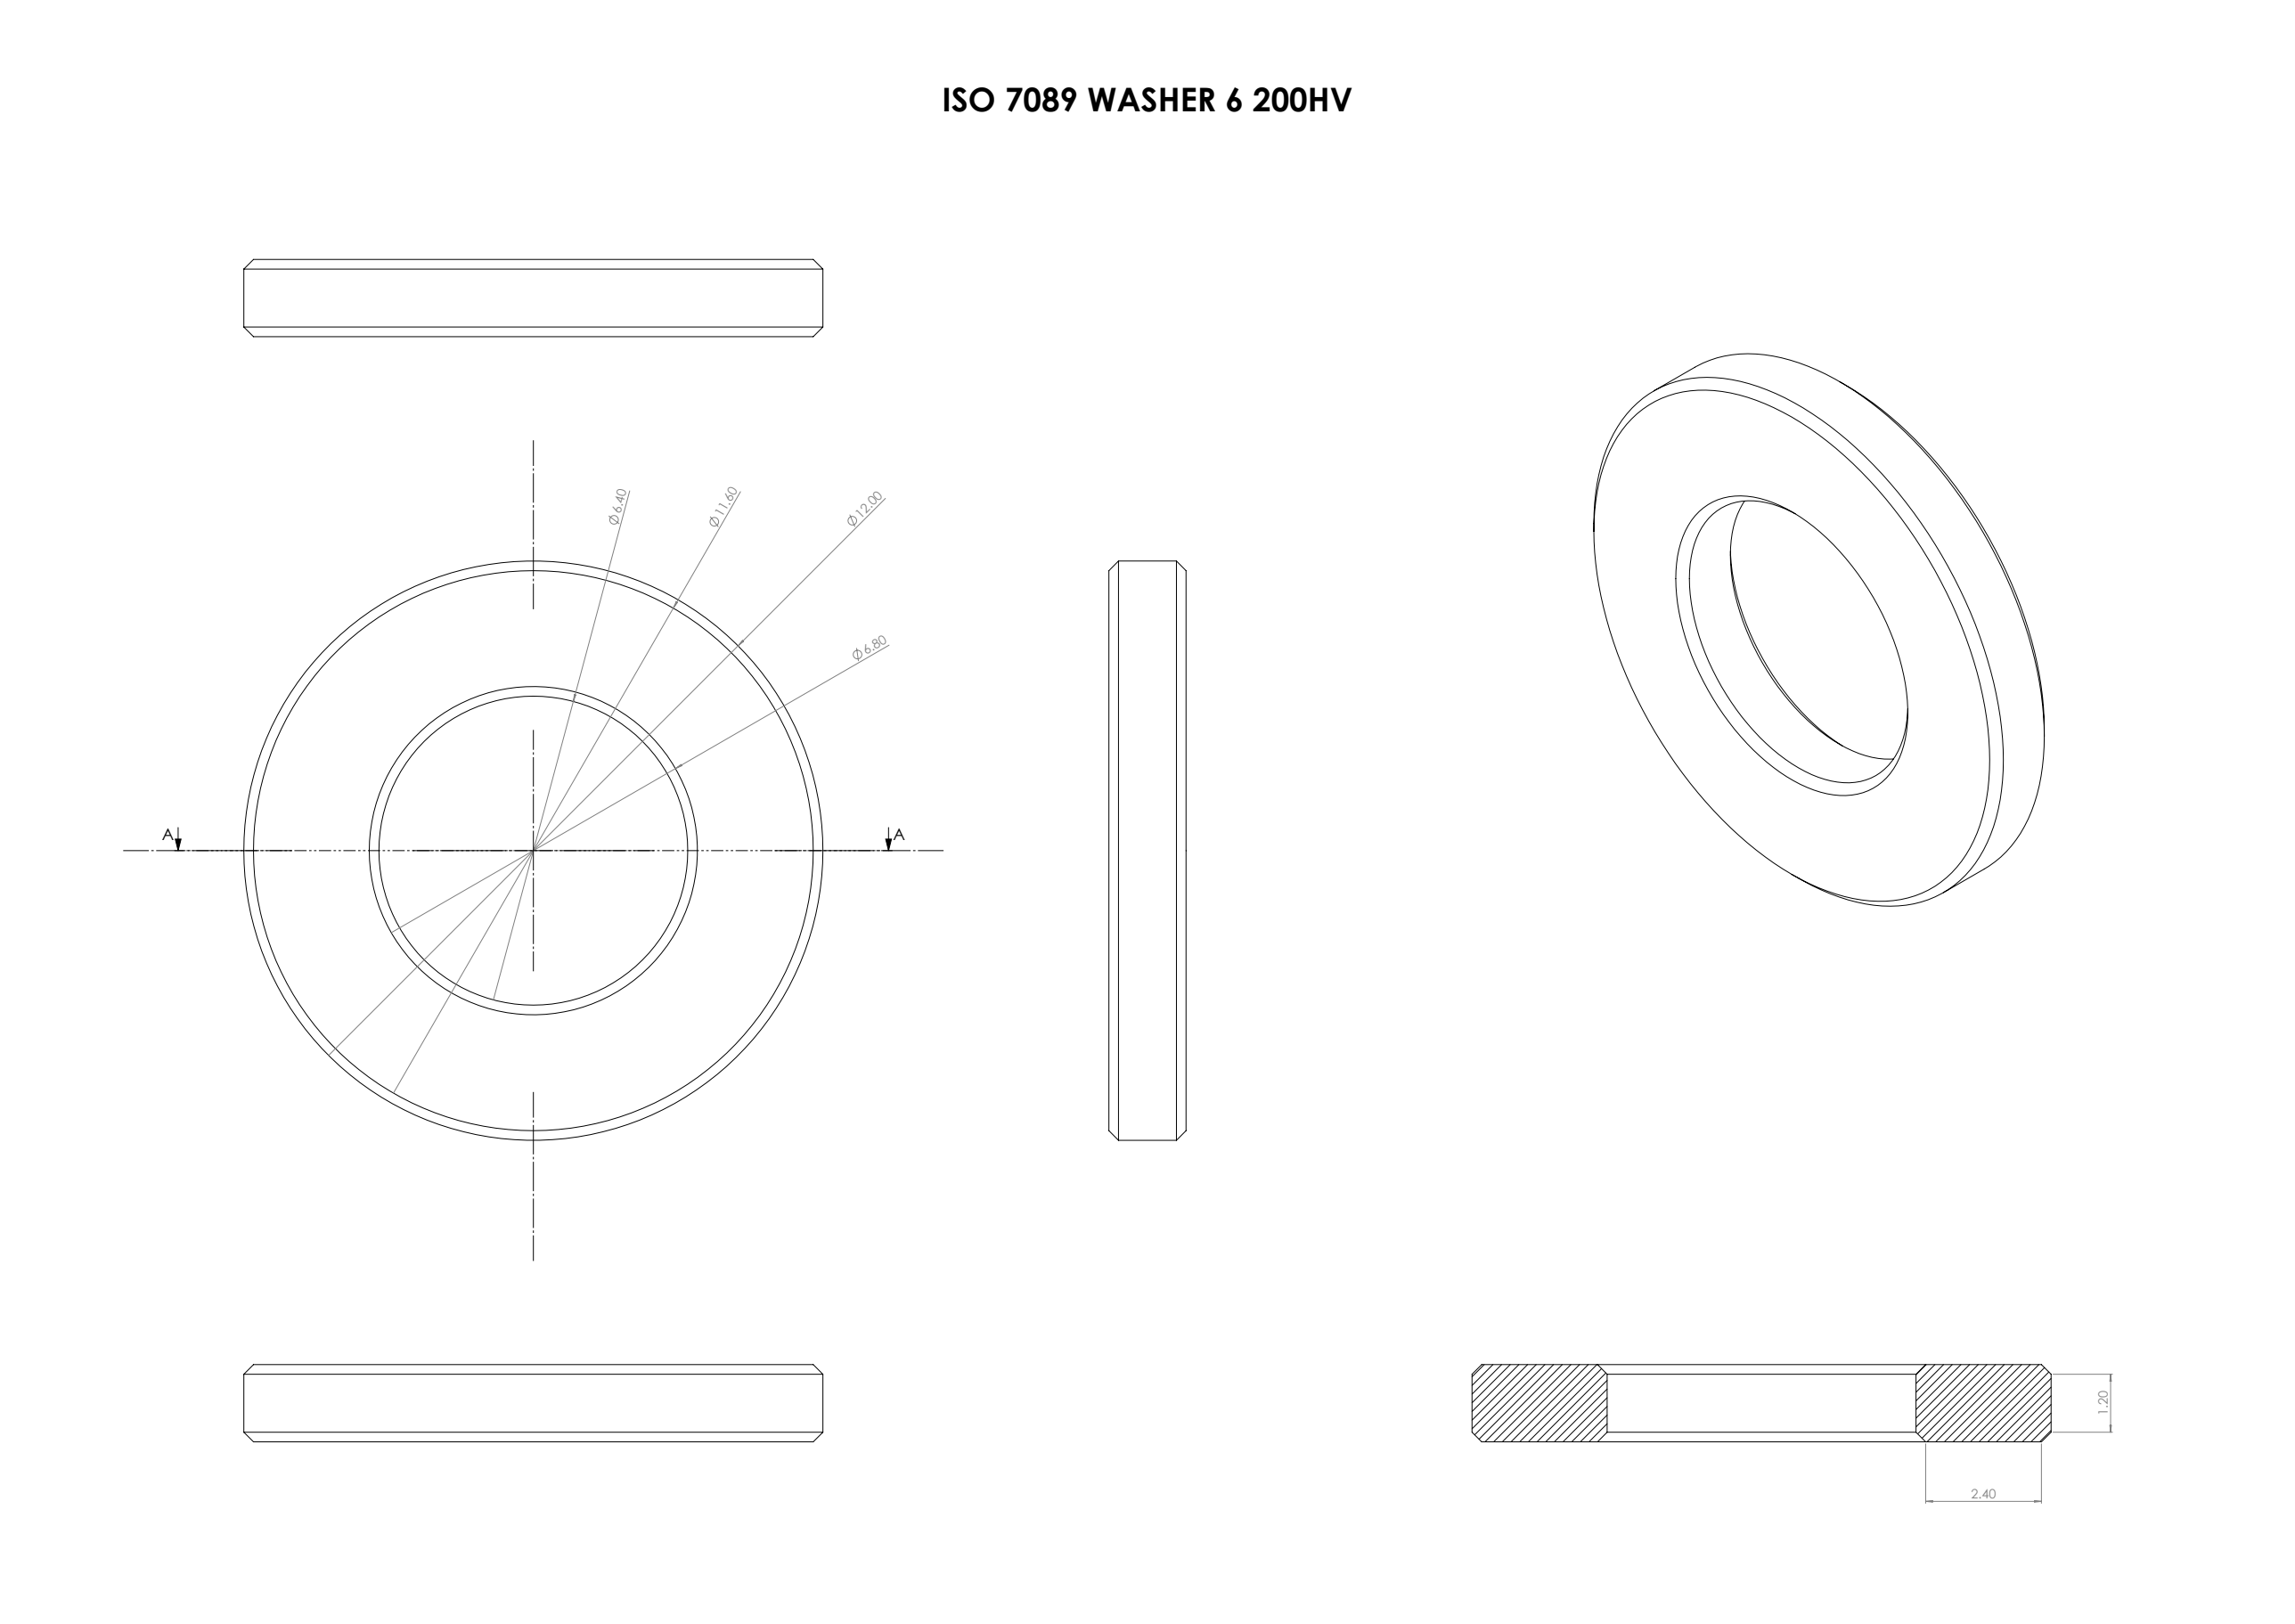
ISO-10303-21;
HEADER;
/* Generated by software containing ST-Developer
 * from STEP Tools, Inc. (www.steptools.com) 
 */

FILE_DESCRIPTION(
/* description */ (''),
/* implementation_level */ '2;1');

FILE_NAME(
/* name */ 
'10_ISO_7089_Washer_6_200HV.step',
/* time_stamp */ '2026-10-22T00:21:42-07:00',
/* author */ (''),
/* organization */ (''),
/* preprocessor_version */ 'ST-DEVELOPER v20.2',
/* originating_system */ 'Autodesk Translation Framework v15.15.0.0',
/* authorisation */ '');

FILE_SCHEMA (('AUTOMOTIVE_DESIGN { 1 0 10303 214 3 1 1 }'));
ENDSEC;

DATA;
#10=MECHANICAL_DESIGN_GEOMETRIC_PRESENTATION_REPRESENTATION('',(#214),#31638);
#192=SHAPE_REPRESENTATION_RELATIONSHIP('SRR','None',#31714,#203);
#203=ADVANCED_BREP_SHAPE_REPRESENTATION('',(#225),#31636);
#214=STYLED_ITEM('',(#31837),#225);
#225=MANIFOLD_SOLID_BREP('Washer',#12489);
#359=CYLINDRICAL_SURFACE('',#13522,0.6);
#360=CYLINDRICAL_SURFACE('',#13528,0.32);
#441=CONICAL_SURFACE('',#13516,0.59,0.785398163397449);
#442=CONICAL_SURFACE('',#13524,0.33,0.785398163397449);
#443=CONICAL_SURFACE('',#13533,0.33,0.785398163397449);
#444=CONICAL_SURFACE('',#13534,0.59,0.785398163397449);
#1401=FACE_BOUND('',#3223,.T.);
#1402=FACE_BOUND('',#3228,.T.);
#1794=CIRCLE('',#13517,0.58);
#1795=CIRCLE('',#13518,0.6);
#1796=CIRCLE('',#13519,0.6);
#1797=CIRCLE('',#13521,0.34);
#1798=CIRCLE('',#13523,0.6);
#1799=CIRCLE('',#13525,0.34);
#1800=CIRCLE('',#13526,0.32);
#1801=CIRCLE('',#13527,0.32);
#1802=CIRCLE('',#13529,0.32);
#1803=CIRCLE('',#13530,0.32);
#1804=CIRCLE('',#13532,0.58);
#2466=FACE_OUTER_BOUND('',#3221,.T.);
#2467=FACE_OUTER_BOUND('',#3222,.T.);
#2468=FACE_OUTER_BOUND('',#3224,.T.);
#2469=FACE_OUTER_BOUND('',#3225,.T.);
#2470=FACE_OUTER_BOUND('',#3226,.T.);
#2471=FACE_OUTER_BOUND('',#3227,.T.);
#2472=FACE_OUTER_BOUND('',#3229,.T.);
#2473=FACE_OUTER_BOUND('',#3230,.T.);
#3221=EDGE_LOOP('',(#11271,#11272,#11273,#11274,#11275));
#3222=EDGE_LOOP('',(#11276));
#3223=EDGE_LOOP('',(#11277));
#3224=EDGE_LOOP('',(#11278,#11279,#11280,#11281,#11282));
#3225=EDGE_LOOP('',(#11283,#11284,#11285,#11286,#11287));
#3226=EDGE_LOOP('',(#11288,#11289,#11290,#11291,#11292,#11293));
#3227=EDGE_LOOP('',(#11294));
#3228=EDGE_LOOP('',(#11295));
#3229=EDGE_LOOP('',(#11296,#11297,#11298,#11299,#11300));
#3230=EDGE_LOOP('',(#11301,#11302,#11303,#11304));
#3946=LINE('',#30956,#4651);
#3947=LINE('',#30965,#4652);
#3948=LINE('',#30971,#4653);
#3949=LINE('',#30980,#4654);
#3950=LINE('',#30985,#4655);
#3951=LINE('',#30987,#4656);
#4651=VECTOR('',#16104,0.59);
#4652=VECTOR('',#16115,0.6);
#4653=VECTOR('',#16122,0.33);
#4654=VECTOR('',#16133,0.32);
#4655=VECTOR('',#16140,0.33);
#4656=VECTOR('',#16143,0.59);
#5825=VERTEX_POINT('',#30953);
#5826=VERTEX_POINT('',#30955);
#5827=VERTEX_POINT('',#30957);
#5828=VERTEX_POINT('',#30961);
#5829=VERTEX_POINT('',#30964);
#5830=VERTEX_POINT('',#30968);
#5831=VERTEX_POINT('',#30970);
#5832=VERTEX_POINT('',#30972);
#5833=VERTEX_POINT('',#30976);
#5834=VERTEX_POINT('',#30977);
#5835=VERTEX_POINT('',#30982);
#7647=EDGE_CURVE('',#5825,#5825,#1794,.T.);
#7648=EDGE_CURVE('',#5825,#5826,#3946,.T.);
#7649=EDGE_CURVE('',#5826,#5827,#1795,.T.);
#7650=EDGE_CURVE('',#5827,#5826,#1796,.T.);
#7651=EDGE_CURVE('',#5828,#5828,#1797,.T.);
#7652=EDGE_CURVE('',#5827,#5829,#3947,.T.);
#7653=EDGE_CURVE('',#5829,#5829,#1798,.T.);
#7654=EDGE_CURVE('',#5830,#5830,#1799,.T.);
#7655=EDGE_CURVE('',#5830,#5831,#3948,.T.);
#7656=EDGE_CURVE('',#5831,#5832,#1800,.T.);
#7657=EDGE_CURVE('',#5832,#5831,#1801,.T.);
#7658=EDGE_CURVE('',#5833,#5834,#1802,.T.);
#7659=EDGE_CURVE('',#5834,#5833,#1803,.T.);
#7660=EDGE_CURVE('',#5834,#5832,#3949,.T.);
#7661=EDGE_CURVE('',#5835,#5835,#1804,.T.);
#7662=EDGE_CURVE('',#5833,#5828,#3950,.T.);
#7663=EDGE_CURVE('',#5829,#5835,#3951,.T.);
#11271=ORIENTED_EDGE('',*,*,#7647,.T.);
#11272=ORIENTED_EDGE('',*,*,#7648,.T.);
#11273=ORIENTED_EDGE('',*,*,#7649,.T.);
#11274=ORIENTED_EDGE('',*,*,#7650,.T.);
#11275=ORIENTED_EDGE('',*,*,#7648,.F.);
#11276=ORIENTED_EDGE('',*,*,#7647,.F.);
#11277=ORIENTED_EDGE('',*,*,#7651,.F.);
#11278=ORIENTED_EDGE('',*,*,#7649,.F.);
#11279=ORIENTED_EDGE('',*,*,#7650,.F.);
#11280=ORIENTED_EDGE('',*,*,#7652,.T.);
#11281=ORIENTED_EDGE('',*,*,#7653,.T.);
#11282=ORIENTED_EDGE('',*,*,#7652,.F.);
#11283=ORIENTED_EDGE('',*,*,#7654,.T.);
#11284=ORIENTED_EDGE('',*,*,#7655,.T.);
#11285=ORIENTED_EDGE('',*,*,#7656,.T.);
#11286=ORIENTED_EDGE('',*,*,#7657,.T.);
#11287=ORIENTED_EDGE('',*,*,#7655,.F.);
#11288=ORIENTED_EDGE('',*,*,#7658,.F.);
#11289=ORIENTED_EDGE('',*,*,#7659,.F.);
#11290=ORIENTED_EDGE('',*,*,#7660,.T.);
#11291=ORIENTED_EDGE('',*,*,#7656,.F.);
#11292=ORIENTED_EDGE('',*,*,#7657,.F.);
#11293=ORIENTED_EDGE('',*,*,#7660,.F.);
#11294=ORIENTED_EDGE('',*,*,#7661,.F.);
#11295=ORIENTED_EDGE('',*,*,#7654,.F.);
#11296=ORIENTED_EDGE('',*,*,#7658,.T.);
#11297=ORIENTED_EDGE('',*,*,#7659,.T.);
#11298=ORIENTED_EDGE('',*,*,#7662,.T.);
#11299=ORIENTED_EDGE('',*,*,#7651,.T.);
#11300=ORIENTED_EDGE('',*,*,#7662,.F.);
#11301=ORIENTED_EDGE('',*,*,#7653,.F.);
#11302=ORIENTED_EDGE('',*,*,#7663,.T.);
#11303=ORIENTED_EDGE('',*,*,#7661,.T.);
#11304=ORIENTED_EDGE('',*,*,#7663,.F.);
#11764=PLANE('',#13520);
#11765=PLANE('',#13531);
#12433=ADVANCED_FACE('',(#2466),#441,.T.);
#12434=ADVANCED_FACE('',(#2467,#1401),#11764,.T.);
#12435=ADVANCED_FACE('',(#2468),#359,.T.);
#12436=ADVANCED_FACE('',(#2469),#442,.F.);
#12437=ADVANCED_FACE('',(#2470),#360,.F.);
#12438=ADVANCED_FACE('',(#2471,#1402),#11765,.T.);
#12439=ADVANCED_FACE('',(#2472),#443,.F.);
#12440=ADVANCED_FACE('',(#2473),#444,.T.);
#12489=CLOSED_SHELL('',(#12433,#12434,#12435,#12436,#12437,#12438,#12439,
#12440));
#13515=AXIS2_PLACEMENT_3D('',#30951,#16098,#16099);
#13516=AXIS2_PLACEMENT_3D('',#30952,#16100,#16101);
#13517=AXIS2_PLACEMENT_3D('',#30954,#16102,#16103);
#13518=AXIS2_PLACEMENT_3D('',#30958,#16105,#16106);
#13519=AXIS2_PLACEMENT_3D('',#30959,#16107,#16108);
#13520=AXIS2_PLACEMENT_3D('',#30960,#16109,#16110);
#13521=AXIS2_PLACEMENT_3D('',#30962,#16111,#16112);
#13522=AXIS2_PLACEMENT_3D('',#30963,#16113,#16114);
#13523=AXIS2_PLACEMENT_3D('',#30966,#16116,#16117);
#13524=AXIS2_PLACEMENT_3D('',#30967,#16118,#16119);
#13525=AXIS2_PLACEMENT_3D('',#30969,#16120,#16121);
#13526=AXIS2_PLACEMENT_3D('',#30973,#16123,#16124);
#13527=AXIS2_PLACEMENT_3D('',#30974,#16125,#16126);
#13528=AXIS2_PLACEMENT_3D('',#30975,#16127,#16128);
#13529=AXIS2_PLACEMENT_3D('',#30978,#16129,#16130);
#13530=AXIS2_PLACEMENT_3D('',#30979,#16131,#16132);
#13531=AXIS2_PLACEMENT_3D('',#30981,#16134,#16135);
#13532=AXIS2_PLACEMENT_3D('',#30983,#16136,#16137);
#13533=AXIS2_PLACEMENT_3D('',#30984,#16138,#16139);
#13534=AXIS2_PLACEMENT_3D('',#30986,#16141,#16142);
#16098=DIRECTION('axis',(0.,0.,1.));
#16099=DIRECTION('refdir',(1.,0.,0.));
#16100=DIRECTION('center_axis',(0.,0.,-1.));
#16101=DIRECTION('ref_axis',(-1.,0.,0.));
#16102=DIRECTION('center_axis',(0.,0.,-1.));
#16103=DIRECTION('ref_axis',(-1.,0.,0.));
#16104=DIRECTION('',(0.707106781186548,8.65956056235494E-17,-0.707106781186547));
#16105=DIRECTION('center_axis',(0.,0.,1.));
#16106=DIRECTION('ref_axis',(-1.,0.,0.));
#16107=DIRECTION('center_axis',(0.,0.,1.));
#16108=DIRECTION('ref_axis',(-1.,0.,0.));
#16109=DIRECTION('center_axis',(0.,0.,1.));
#16110=DIRECTION('ref_axis',(1.,0.,0.));
#16111=DIRECTION('center_axis',(0.,0.,1.));
#16112=DIRECTION('ref_axis',(-1.,0.,0.));
#16113=DIRECTION('center_axis',(0.,0.,1.));
#16114=DIRECTION('ref_axis',(1.,0.,0.));
#16115=DIRECTION('',(0.,0.,-1.));
#16116=DIRECTION('center_axis',(0.,0.,1.));
#16117=DIRECTION('ref_axis',(1.,0.,0.));
#16118=DIRECTION('center_axis',(0.,0.,-1.));
#16119=DIRECTION('ref_axis',(-1.,0.,0.));
#16120=DIRECTION('center_axis',(0.,0.,-1.));
#16121=DIRECTION('ref_axis',(-1.,0.,0.));
#16122=DIRECTION('',(-0.707106781186548,8.65956056235494E-17,0.707106781186547));
#16123=DIRECTION('center_axis',(0.,0.,1.));
#16124=DIRECTION('ref_axis',(-1.,0.,0.));
#16125=DIRECTION('center_axis',(0.,0.,1.));
#16126=DIRECTION('ref_axis',(-1.,0.,0.));
#16127=DIRECTION('center_axis',(0.,0.,1.));
#16128=DIRECTION('ref_axis',(1.,0.,0.));
#16129=DIRECTION('center_axis',(0.,0.,-1.));
#16130=DIRECTION('ref_axis',(-1.,0.,0.));
#16131=DIRECTION('center_axis',(0.,0.,-1.));
#16132=DIRECTION('ref_axis',(-1.,0.,0.));
#16133=DIRECTION('',(0.,0.,-1.));
#16134=DIRECTION('center_axis',(0.,0.,-1.));
#16135=DIRECTION('ref_axis',(-1.,0.,0.));
#16136=DIRECTION('center_axis',(0.,0.,1.));
#16137=DIRECTION('ref_axis',(1.,0.,0.));
#16138=DIRECTION('center_axis',(0.,0.,1.));
#16139=DIRECTION('ref_axis',(-1.,0.,0.));
#16140=DIRECTION('',(0.707106781186548,-8.65956056235494E-17,0.707106781186547));
#16141=DIRECTION('center_axis',(0.,0.,1.));
#16142=DIRECTION('ref_axis',(1.,0.,0.));
#16143=DIRECTION('',(0.707106781186548,8.65956056235494E-17,-0.707106781186547));
#30951=CARTESIAN_POINT('',(0.,0.,0.));
#30952=CARTESIAN_POINT('Origin',(0.,0.,0.15));
#30953=CARTESIAN_POINT('',(0.58,-7.10295143505465E-17,0.16));
#30954=CARTESIAN_POINT('Origin',(0.,0.,0.16));
#30955=CARTESIAN_POINT('',(0.6,7.34788079488412E-17,0.14));
#30956=CARTESIAN_POINT('',(0.59,7.22541611496938E-17,0.15));
#30957=CARTESIAN_POINT('',(-0.6,-7.34788079488412E-17,0.14));
#30958=CARTESIAN_POINT('Origin',(0.,0.,0.14));
#30959=CARTESIAN_POINT('Origin',(0.,0.,0.14));
#30960=CARTESIAN_POINT('Origin',(0.32,0.,0.16));
#30961=CARTESIAN_POINT('',(0.34,4.163799117101E-17,0.16));
#30962=CARTESIAN_POINT('Origin',(0.,0.,0.16));
#30963=CARTESIAN_POINT('Origin',(0.,0.,0.09));
#30964=CARTESIAN_POINT('',(-0.6,-7.34788079488412E-17,0.02));
#30965=CARTESIAN_POINT('',(-0.6,-7.34788079488412E-17,0.09));
#30966=CARTESIAN_POINT('Origin',(0.,0.,0.02));
#30967=CARTESIAN_POINT('Origin',(0.,0.,0.01));
#30968=CARTESIAN_POINT('',(0.34,-4.163799117101E-17,0.));
#30969=CARTESIAN_POINT('Origin',(0.,0.,0.));
#30970=CARTESIAN_POINT('',(0.32,3.91886975727153E-17,0.02));
#30971=CARTESIAN_POINT('',(0.33,-4.04133443718627E-17,0.01));
#30972=CARTESIAN_POINT('',(-0.32,-3.91886975727153E-17,0.02));
#30973=CARTESIAN_POINT('Origin',(0.,0.,0.02));
#30974=CARTESIAN_POINT('Origin',(0.,0.,0.02));
#30975=CARTESIAN_POINT('Origin',(0.,0.,0.08));
#30976=CARTESIAN_POINT('',(0.32,-3.91886975727153E-17,0.14));
#30977=CARTESIAN_POINT('',(-0.32,-3.91886975727153E-17,0.14));
#30978=CARTESIAN_POINT('Origin',(0.,0.,0.14));
#30979=CARTESIAN_POINT('Origin',(0.,0.,0.14));
#30980=CARTESIAN_POINT('',(-0.32,-3.91886975727153E-17,0.08));
#30981=CARTESIAN_POINT('Origin',(0.58,0.,0.));
#30982=CARTESIAN_POINT('',(-0.58,-7.10295143505465E-17,-1.73472347597681E-18));
#30983=CARTESIAN_POINT('Origin',(0.,0.,0.));
#30984=CARTESIAN_POINT('Origin',(0.,0.,0.15));
#30985=CARTESIAN_POINT('',(0.33,-4.04133443718627E-17,0.15));
#30986=CARTESIAN_POINT('Origin',(0.,0.,0.01));
#30987=CARTESIAN_POINT('',(-0.59,-7.22541611496938E-17,0.01));
#31623=UNCERTAINTY_MEASURE_WITH_UNIT(LENGTH_MEASURE(0.001),#31639,
'DISTANCE_ACCURACY_VALUE',
'Maximum model space distance between geometric entities at asserted c
onnectivities');
#31625=UNCERTAINTY_MEASURE_WITH_UNIT(LENGTH_MEASURE(0.001),#31639,
'DISTANCE_ACCURACY_VALUE',
'Maximum model space distance between geometric entities at asserted c
onnectivities');
#31636=(
GEOMETRIC_REPRESENTATION_CONTEXT(3)
GLOBAL_UNCERTAINTY_ASSIGNED_CONTEXT((#31623))
GLOBAL_UNIT_ASSIGNED_CONTEXT((#31639,#31641,#31642))
REPRESENTATION_CONTEXT('','3D')
);
#31638=(
GEOMETRIC_REPRESENTATION_CONTEXT(3)
GLOBAL_UNCERTAINTY_ASSIGNED_CONTEXT((#31625))
GLOBAL_UNIT_ASSIGNED_CONTEXT((#31639,#31641,#31642))
REPRESENTATION_CONTEXT('','3D')
);
#31639=(
LENGTH_UNIT()
NAMED_UNIT(*)
SI_UNIT(.CENTI.,.METRE.)
);
#31641=(
NAMED_UNIT(*)
PLANE_ANGLE_UNIT()
SI_UNIT($,.RADIAN.)
);
#31642=(
NAMED_UNIT(*)
SI_UNIT($,.STERADIAN.)
SOLID_ANGLE_UNIT()
);
#31653=SHAPE_DEFINITION_REPRESENTATION(#31665,#31714);
#31665=PRODUCT_DEFINITION_SHAPE('',$,#31727);
#31714=SHAPE_REPRESENTATION('',(#13515),#31636);
#31716=PRODUCT_DEFINITION_CONTEXT('part definition',#31754,'design');
#31727=PRODUCT_DEFINITION('2026-10-22-02-42-33-064',
'10_ISO_7089_Washer_6_200HV',#31739,#31716);
#31739=PRODUCT_DEFINITION_FORMATION('',$,#31766);
#31754=APPLICATION_CONTEXT(
'Core Data for Automotive Mechanical Design Process');
#31755=PRODUCT_CONTEXT('part definition',#31754,'mechanical');
#31766=PRODUCT('2026-10-22-02-42-33-064','10_ISO_7089_Washer_6_200HV',$,
(#31755));
#31831=COLOUR_RGB('Black',0.12,0.14,0.17);
#31832=FILL_AREA_STYLE_COLOUR('',#31831);
#31833=FILL_AREA_STYLE('',(#31832));
#31834=SURFACE_STYLE_FILL_AREA(#31833);
#31835=SURFACE_SIDE_STYLE('',(#31834));
#31836=SURFACE_STYLE_USAGE(.BOTH.,#31835);
#31837=PRESENTATION_STYLE_ASSIGNMENT((#31836));
ENDSEC;
END-ISO-10303-21;
